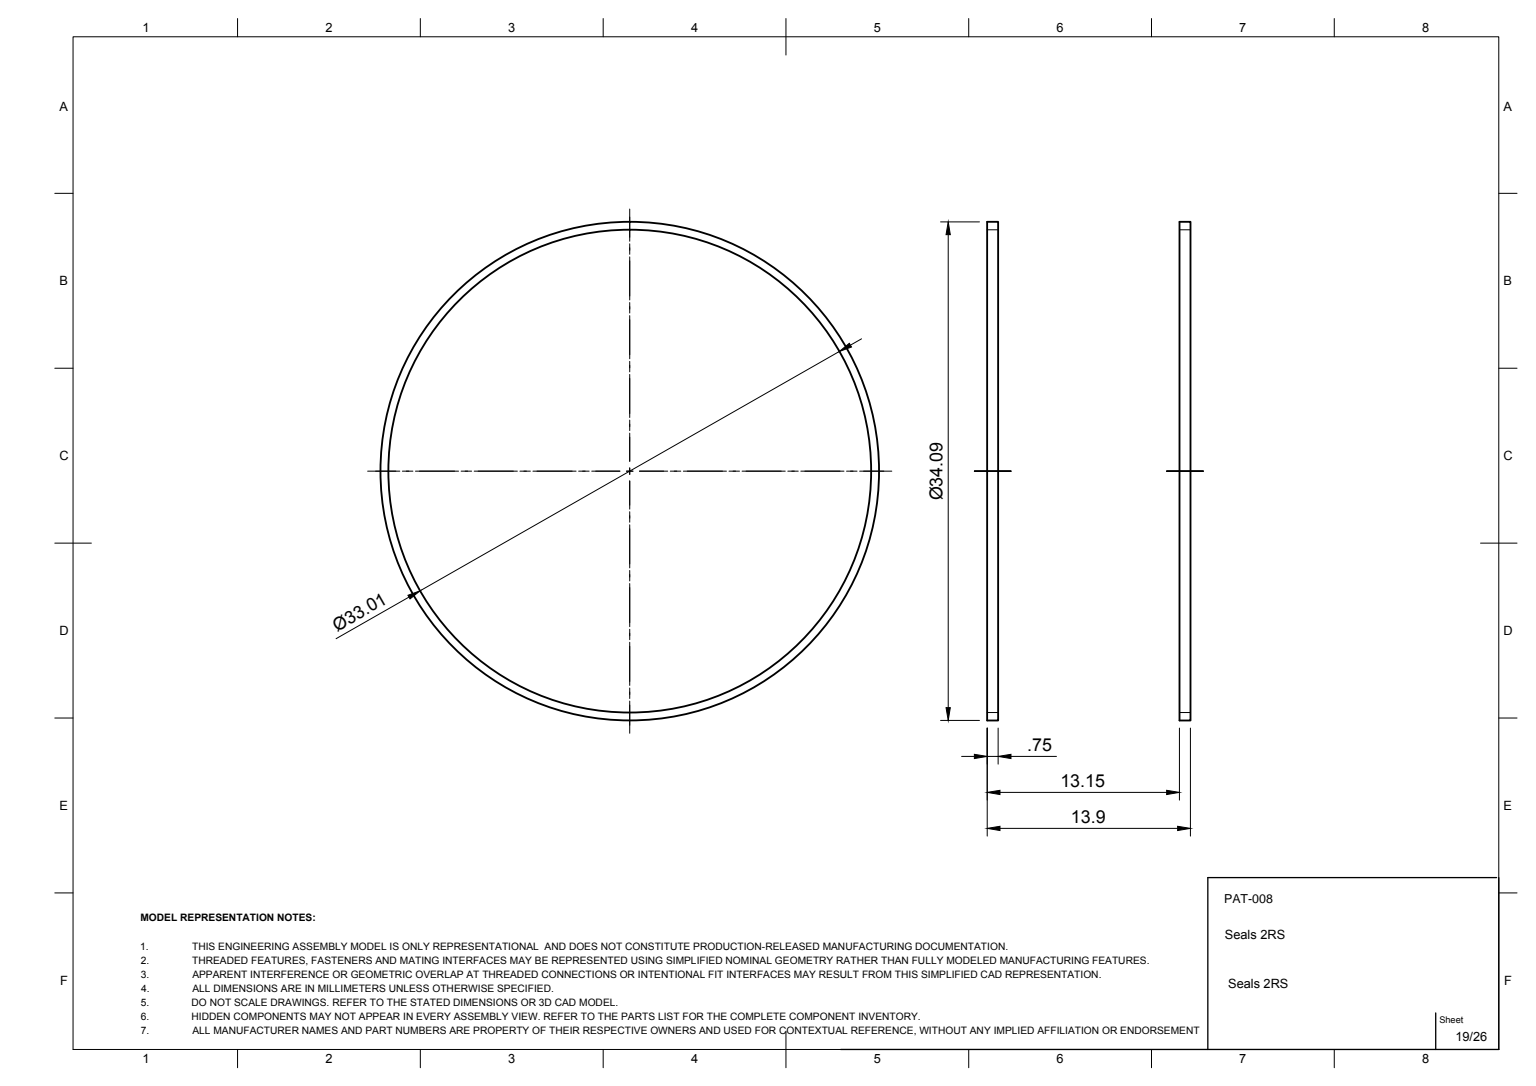
ISO-10303-21;
HEADER;
/* Generated by software containing ST-Developer
 * from STEP Tools, Inc. (www.steptools.com) 
 */

FILE_DESCRIPTION(
/* description */ ('Bearing housing with oil seal and end cap'),
/* implementation_level */ '2;1');

FILE_NAME(
/* name */ 'Seals 2RS.step',
/* time_stamp */ '2026-10-28T03:23:10-07:00',
/* author */ (''),
/* organization */ (''),
/* preprocessor_version */ 'ST-DEVELOPER v20.2',
/* originating_system */ 'Autodesk Translation Framework v15.17.0.0',
/* authorisation */ '');

FILE_SCHEMA (('AUTOMOTIVE_DESIGN { 1 0 10303 214 3 1 1 }'));
ENDSEC;

DATA;
#10=MECHANICAL_DESIGN_GEOMETRIC_PRESENTATION_REPRESENTATION('',(#278,#279),#7871);
#229=SHAPE_REPRESENTATION_RELATIONSHIP('SRR','None',#7977,#250);
#250=ADVANCED_BREP_SHAPE_REPRESENTATION('',(#307,#308),#7861);
#278=STYLED_ITEM('',(#8153),#307);
#279=STYLED_ITEM('',(#8153),#308);
#307=MANIFOLD_SOLID_BREP('Body1',#4104);
#308=MANIFOLD_SOLID_BREP('Body2',#4105);
#379=FACE_BOUND('',#1016,.T.);
#380=FACE_BOUND('',#1019,.T.);
#381=FACE_BOUND('',#1022,.T.);
#382=FACE_BOUND('',#1025,.T.);
#484=PLANE('',#4668);
#485=PLANE('',#4673);
#486=PLANE('',#4676);
#487=PLANE('',#4681);
#700=FACE_OUTER_BOUND('',#1015,.T.);
#701=FACE_OUTER_BOUND('',#1017,.T.);
#702=FACE_OUTER_BOUND('',#1018,.T.);
#703=FACE_OUTER_BOUND('',#1020,.T.);
#704=FACE_OUTER_BOUND('',#1021,.T.);
#705=FACE_OUTER_BOUND('',#1023,.T.);
#706=FACE_OUTER_BOUND('',#1024,.T.);
#707=FACE_OUTER_BOUND('',#1026,.T.);
#1015=EDGE_LOOP('',(#3343));
#1016=EDGE_LOOP('',(#3344));
#1017=EDGE_LOOP('',(#3345,#3346,#3347,#3348));
#1018=EDGE_LOOP('',(#3349));
#1019=EDGE_LOOP('',(#3350));
#1020=EDGE_LOOP('',(#3351,#3352,#3353,#3354));
#1021=EDGE_LOOP('',(#3355));
#1022=EDGE_LOOP('',(#3356));
#1023=EDGE_LOOP('',(#3357,#3358,#3359,#3360));
#1024=EDGE_LOOP('',(#3361));
#1025=EDGE_LOOP('',(#3362));
#1026=EDGE_LOOP('',(#3363,#3364,#3365,#3366));
#1273=LINE('',#7224,#1535);
#1274=LINE('',#7229,#1536);
#1275=LINE('',#7238,#1537);
#1276=LINE('',#7243,#1538);
#1535=VECTOR('',#5656,1.70469);
#1536=VECTOR('',#5663,1.65031);
#1537=VECTOR('',#5674,1.70469);
#1538=VECTOR('',#5681,1.65031);
#1827=CIRCLE('',#4669,1.70469);
#1828=CIRCLE('',#4670,1.65031);
#1829=CIRCLE('',#4672,1.70469);
#1830=CIRCLE('',#4674,1.65031);
#1831=CIRCLE('',#4677,1.70469);
#1832=CIRCLE('',#4678,1.65031);
#1833=CIRCLE('',#4680,1.70469);
#1834=CIRCLE('',#4682,1.65031);
#2099=VERTEX_POINT('',#7217);
#2100=VERTEX_POINT('',#7219);
#2101=VERTEX_POINT('',#7222);
#2102=VERTEX_POINT('',#7226);
#2103=VERTEX_POINT('',#7231);
#2104=VERTEX_POINT('',#7233);
#2105=VERTEX_POINT('',#7236);
#2106=VERTEX_POINT('',#7240);
#2535=EDGE_CURVE('',#2099,#2099,#1827,.T.);
#2536=EDGE_CURVE('',#2100,#2100,#1828,.T.);
#2537=EDGE_CURVE('',#2101,#2101,#1829,.T.);
#2538=EDGE_CURVE('',#2101,#2099,#1273,.T.);
#2539=EDGE_CURVE('',#2102,#2102,#1830,.T.);
#2540=EDGE_CURVE('',#2102,#2100,#1274,.T.);
#2541=EDGE_CURVE('',#2103,#2103,#1831,.T.);
#2542=EDGE_CURVE('',#2104,#2104,#1832,.T.);
#2543=EDGE_CURVE('',#2105,#2105,#1833,.T.);
#2544=EDGE_CURVE('',#2105,#2103,#1275,.T.);
#2545=EDGE_CURVE('',#2106,#2106,#1834,.T.);
#2546=EDGE_CURVE('',#2106,#2104,#1276,.T.);
#3343=ORIENTED_EDGE('',*,*,#2535,.F.);
#3344=ORIENTED_EDGE('',*,*,#2536,.T.);
#3345=ORIENTED_EDGE('',*,*,#2537,.F.);
#3346=ORIENTED_EDGE('',*,*,#2538,.T.);
#3347=ORIENTED_EDGE('',*,*,#2535,.T.);
#3348=ORIENTED_EDGE('',*,*,#2538,.F.);
#3349=ORIENTED_EDGE('',*,*,#2537,.T.);
#3350=ORIENTED_EDGE('',*,*,#2539,.F.);
#3351=ORIENTED_EDGE('',*,*,#2539,.T.);
#3352=ORIENTED_EDGE('',*,*,#2540,.T.);
#3353=ORIENTED_EDGE('',*,*,#2536,.F.);
#3354=ORIENTED_EDGE('',*,*,#2540,.F.);
#3355=ORIENTED_EDGE('',*,*,#2541,.F.);
#3356=ORIENTED_EDGE('',*,*,#2542,.T.);
#3357=ORIENTED_EDGE('',*,*,#2543,.F.);
#3358=ORIENTED_EDGE('',*,*,#2544,.T.);
#3359=ORIENTED_EDGE('',*,*,#2541,.T.);
#3360=ORIENTED_EDGE('',*,*,#2544,.F.);
#3361=ORIENTED_EDGE('',*,*,#2543,.T.);
#3362=ORIENTED_EDGE('',*,*,#2545,.F.);
#3363=ORIENTED_EDGE('',*,*,#2545,.T.);
#3364=ORIENTED_EDGE('',*,*,#2546,.T.);
#3365=ORIENTED_EDGE('',*,*,#2542,.F.);
#3366=ORIENTED_EDGE('',*,*,#2546,.F.);
#3809=CYLINDRICAL_SURFACE('',#4671,1.70469);
#3810=CYLINDRICAL_SURFACE('',#4675,1.65031);
#3811=CYLINDRICAL_SURFACE('',#4679,1.70469);
#3812=CYLINDRICAL_SURFACE('',#4683,1.65031);
#3982=ADVANCED_FACE('',(#700,#379),#484,.T.);
#3983=ADVANCED_FACE('',(#701),#3809,.T.);
#3984=ADVANCED_FACE('',(#702,#380),#485,.T.);
#3985=ADVANCED_FACE('',(#703),#3810,.F.);
#3986=ADVANCED_FACE('',(#704,#381),#486,.T.);
#3987=ADVANCED_FACE('',(#705),#3811,.T.);
#3988=ADVANCED_FACE('',(#706,#382),#487,.T.);
#3989=ADVANCED_FACE('',(#707),#3812,.F.);
#4104=CLOSED_SHELL('',(#3982,#3983,#3984,#3985));
#4105=CLOSED_SHELL('',(#3986,#3987,#3988,#3989));
#4667=AXIS2_PLACEMENT_3D('',#7215,#5644,#5645);
#4668=AXIS2_PLACEMENT_3D('',#7216,#5646,#5647);
#4669=AXIS2_PLACEMENT_3D('',#7218,#5648,#5649);
#4670=AXIS2_PLACEMENT_3D('',#7220,#5650,#5651);
#4671=AXIS2_PLACEMENT_3D('',#7221,#5652,#5653);
#4672=AXIS2_PLACEMENT_3D('',#7223,#5654,#5655);
#4673=AXIS2_PLACEMENT_3D('',#7225,#5657,#5658);
#4674=AXIS2_PLACEMENT_3D('',#7227,#5659,#5660);
#4675=AXIS2_PLACEMENT_3D('',#7228,#5661,#5662);
#4676=AXIS2_PLACEMENT_3D('',#7230,#5664,#5665);
#4677=AXIS2_PLACEMENT_3D('',#7232,#5666,#5667);
#4678=AXIS2_PLACEMENT_3D('',#7234,#5668,#5669);
#4679=AXIS2_PLACEMENT_3D('',#7235,#5670,#5671);
#4680=AXIS2_PLACEMENT_3D('',#7237,#5672,#5673);
#4681=AXIS2_PLACEMENT_3D('',#7239,#5675,#5676);
#4682=AXIS2_PLACEMENT_3D('',#7241,#5677,#5678);
#4683=AXIS2_PLACEMENT_3D('',#7242,#5679,#5680);
#5644=DIRECTION('axis',(0.,0.,1.));
#5645=DIRECTION('refdir',(1.,0.,0.));
#5646=DIRECTION('center_axis',(0.,1.,0.));
#5647=DIRECTION('ref_axis',(0.,0.,1.));
#5648=DIRECTION('center_axis',(0.,-1.,0.));
#5649=DIRECTION('ref_axis',(1.,0.,0.));
#5650=DIRECTION('center_axis',(0.,-1.,0.));
#5651=DIRECTION('ref_axis',(1.,0.,0.));
#5652=DIRECTION('center_axis',(0.,-1.,0.));
#5653=DIRECTION('ref_axis',(1.,0.,0.));
#5654=DIRECTION('center_axis',(0.,-1.,0.));
#5655=DIRECTION('ref_axis',(1.,0.,0.));
#5656=DIRECTION('',(0.,1.,0.));
#5657=DIRECTION('center_axis',(0.,-1.,0.));
#5658=DIRECTION('ref_axis',(0.,0.,-1.));
#5659=DIRECTION('center_axis',(0.,-1.,0.));
#5660=DIRECTION('ref_axis',(1.,0.,0.));
#5661=DIRECTION('center_axis',(0.,-1.,0.));
#5662=DIRECTION('ref_axis',(1.,0.,0.));
#5663=DIRECTION('',(0.,1.,0.));
#5664=DIRECTION('center_axis',(0.,1.,0.));
#5665=DIRECTION('ref_axis',(0.,0.,1.));
#5666=DIRECTION('center_axis',(0.,-1.,0.));
#5667=DIRECTION('ref_axis',(1.,0.,0.));
#5668=DIRECTION('center_axis',(0.,-1.,0.));
#5669=DIRECTION('ref_axis',(1.,0.,0.));
#5670=DIRECTION('center_axis',(0.,-1.,0.));
#5671=DIRECTION('ref_axis',(1.,0.,0.));
#5672=DIRECTION('center_axis',(0.,-1.,0.));
#5673=DIRECTION('ref_axis',(1.,0.,0.));
#5674=DIRECTION('',(0.,1.,0.));
#5675=DIRECTION('center_axis',(0.,-1.,0.));
#5676=DIRECTION('ref_axis',(0.,0.,-1.));
#5677=DIRECTION('center_axis',(0.,-1.,0.));
#5678=DIRECTION('ref_axis',(1.,0.,0.));
#5679=DIRECTION('center_axis',(0.,-1.,0.));
#5680=DIRECTION('ref_axis',(1.,0.,0.));
#5681=DIRECTION('',(0.,1.,0.));
#7215=CARTESIAN_POINT('',(0.,0.,0.));
#7216=CARTESIAN_POINT('Origin',(1.70469,0.695,0.));
#7217=CARTESIAN_POINT('',(-1.70469,0.695,-2.0876431520385E-16));
#7218=CARTESIAN_POINT('Origin',(0.,0.695,0.));
#7219=CARTESIAN_POINT('',(-1.65031,0.695,-2.02104685910087E-16));
#7220=CARTESIAN_POINT('Origin',(0.,0.695,0.));
#7221=CARTESIAN_POINT('Origin',(0.,0.6575,0.));
#7222=CARTESIAN_POINT('',(-1.70469,0.62,-2.0876431520385E-16));
#7223=CARTESIAN_POINT('Origin',(0.,0.62,0.));
#7224=CARTESIAN_POINT('',(-1.70469,0.6575,-2.0876431520385E-16));
#7225=CARTESIAN_POINT('Origin',(1.65031,0.62,0.));
#7226=CARTESIAN_POINT('',(-1.65031,0.62,-2.02104685910087E-16));
#7227=CARTESIAN_POINT('Origin',(0.,0.62,0.));
#7228=CARTESIAN_POINT('Origin',(0.,0.6575,0.));
#7229=CARTESIAN_POINT('',(-1.65031,0.6575,-2.02104685910087E-16));
#7230=CARTESIAN_POINT('Origin',(1.70469,-0.62,0.));
#7231=CARTESIAN_POINT('',(-1.70469,-0.62,-2.0876431520385E-16));
#7232=CARTESIAN_POINT('Origin',(0.,-0.62,0.));
#7233=CARTESIAN_POINT('',(-1.65031,-0.62,-2.02104685910087E-16));
#7234=CARTESIAN_POINT('Origin',(0.,-0.62,0.));
#7235=CARTESIAN_POINT('Origin',(0.,-0.6575,0.));
#7236=CARTESIAN_POINT('',(-1.70469,-0.695,-2.0876431520385E-16));
#7237=CARTESIAN_POINT('Origin',(0.,-0.695,0.));
#7238=CARTESIAN_POINT('',(-1.70469,-0.6575,-2.0876431520385E-16));
#7239=CARTESIAN_POINT('Origin',(1.65031,-0.695,0.));
#7240=CARTESIAN_POINT('',(-1.65031,-0.695,-2.02104685910087E-16));
#7241=CARTESIAN_POINT('Origin',(0.,-0.695,0.));
#7242=CARTESIAN_POINT('Origin',(0.,-0.6575,0.));
#7243=CARTESIAN_POINT('',(-1.65031,-0.6575,-2.02104685910087E-16));
#7835=UNCERTAINTY_MEASURE_WITH_UNIT(LENGTH_MEASURE(0.001),#7872,
'DISTANCE_ACCURACY_VALUE',
'Maximum model space distance between geometric entities at asserted c
onnectivities');
#7845=UNCERTAINTY_MEASURE_WITH_UNIT(LENGTH_MEASURE(0.001),#7872,
'DISTANCE_ACCURACY_VALUE',
'Maximum model space distance between geometric entities at asserted c
onnectivities');
#7861=(
GEOMETRIC_REPRESENTATION_CONTEXT(3)
GLOBAL_UNCERTAINTY_ASSIGNED_CONTEXT((#7835))
GLOBAL_UNIT_ASSIGNED_CONTEXT((#7872,#7874,#7875))
REPRESENTATION_CONTEXT('','3D')
);
#7871=(
GEOMETRIC_REPRESENTATION_CONTEXT(3)
GLOBAL_UNCERTAINTY_ASSIGNED_CONTEXT((#7845))
GLOBAL_UNIT_ASSIGNED_CONTEXT((#7872,#7874,#7875))
REPRESENTATION_CONTEXT('','3D')
);
#7872=(
LENGTH_UNIT()
NAMED_UNIT(*)
SI_UNIT(.CENTI.,.METRE.)
);
#7874=(
NAMED_UNIT(*)
PLANE_ANGLE_UNIT()
SI_UNIT($,.RADIAN.)
);
#7875=(
NAMED_UNIT(*)
SI_UNIT($,.STERADIAN.)
SOLID_ANGLE_UNIT()
);
#7891=SHAPE_DEFINITION_REPRESENTATION(#7916,#7977);
#7916=PRODUCT_DEFINITION_SHAPE('',$,#8003);
#7977=SHAPE_REPRESENTATION('',(#4667),#7861);
#7987=PRODUCT_DEFINITION_CONTEXT('part definition',#8064,'design');
#8003=PRODUCT_DEFINITION('Seals 2RS','Seals 2RS',#8028,#7987);
#8028=PRODUCT_DEFINITION_FORMATION('',$,#8081);
#8064=APPLICATION_CONTEXT(
'Core Data for Automotive Mechanical Design Process');
#8065=PRODUCT_CONTEXT('part definition',#8064,'mechanical');
#8081=PRODUCT('Seals 2RS','Seals 2RS','Seals 2RS',(#8065));
#8147=COLOUR_RGB('Grey',0.48,0.52,0.57);
#8148=FILL_AREA_STYLE_COLOUR('',#8147);
#8149=FILL_AREA_STYLE('',(#8148));
#8150=SURFACE_STYLE_FILL_AREA(#8149);
#8151=SURFACE_SIDE_STYLE('',(#8150));
#8152=SURFACE_STYLE_USAGE(.BOTH.,#8151);
#8153=PRESENTATION_STYLE_ASSIGNMENT((#8152));
ENDSEC;
END-ISO-10303-21;
